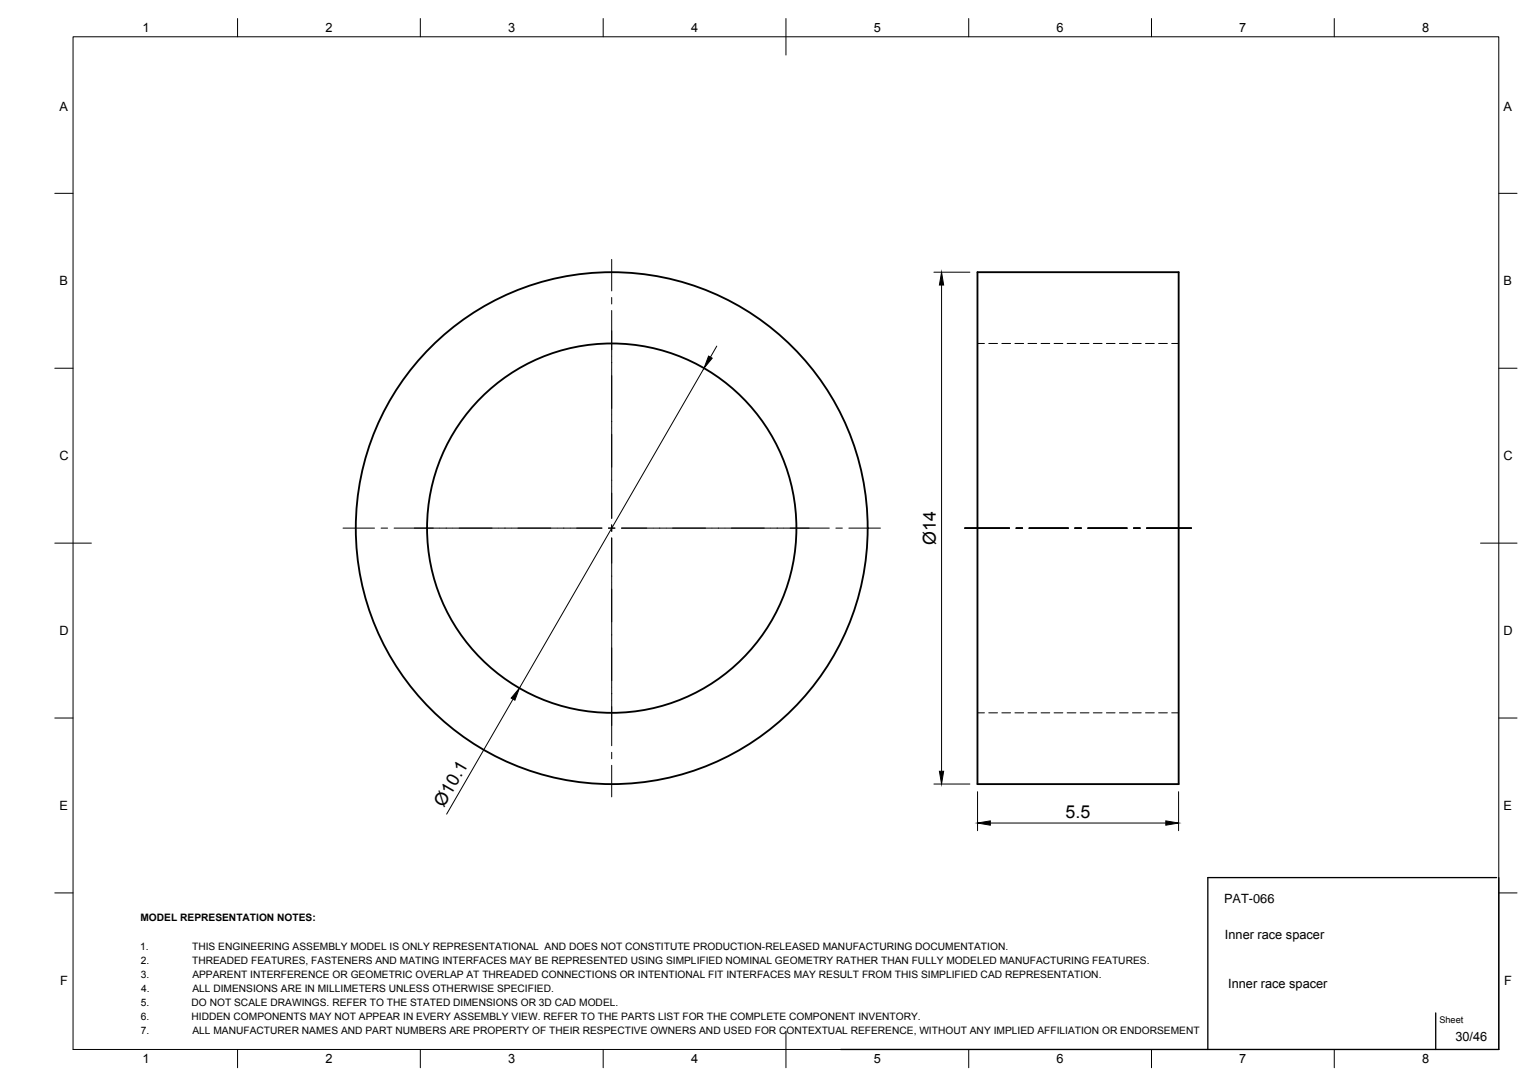
ISO-10303-21;
HEADER;
/* Generated by software containing ST-Developer
 * from STEP Tools, Inc. (www.steptools.com) 
 */

FILE_DESCRIPTION(
/* description */ ('Lever-operated bar clamp (toggle)'),
/* implementation_level */ '2;1');

FILE_NAME(
/* name */ 'Inner race spacer.step',
/* time_stamp */ '2026-10-28T03:25:02-07:00',
/* author */ (''),
/* organization */ (''),
/* preprocessor_version */ 'ST-DEVELOPER v20.2',
/* originating_system */ 'Autodesk Translation Framework v15.17.0.0',
/* authorisation */ '');

FILE_SCHEMA (('AUTOMOTIVE_DESIGN { 1 0 10303 214 3 1 1 }'));
ENDSEC;

DATA;
#10=MECHANICAL_DESIGN_GEOMETRIC_PRESENTATION_REPRESENTATION('',(#439),#12413);
#355=SHAPE_REPRESENTATION_RELATIONSHIP('SRR','None',#12597,#393);
#393=ADVANCED_BREP_SHAPE_REPRESENTATION('',(#484),#12394);
#439=STYLED_ITEM('',(#12869),#484);
#484=MANIFOLD_SOLID_BREP('Body1',#6600);
#615=FACE_BOUND('',#1676,.T.);
#616=FACE_BOUND('',#1678,.T.);
#796=PLANE('',#7588);
#797=PLANE('',#7589);
#1152=FACE_OUTER_BOUND('',#1673,.T.);
#1153=FACE_OUTER_BOUND('',#1674,.T.);
#1154=FACE_OUTER_BOUND('',#1675,.T.);
#1155=FACE_OUTER_BOUND('',#1677,.T.);
#1673=EDGE_LOOP('',(#5501,#5502,#5503,#5504));
#1674=EDGE_LOOP('',(#5505,#5506,#5507,#5508));
#1675=EDGE_LOOP('',(#5509));
#1676=EDGE_LOOP('',(#5510));
#1677=EDGE_LOOP('',(#5511));
#1678=EDGE_LOOP('',(#5512));
#2128=LINE('',#11592,#2569);
#2129=LINE('',#11598,#2570);
#2569=VECTOR('',#9261,0.505);
#2570=VECTOR('',#9268,0.7);
#2978=CIRCLE('',#7583,0.505);
#2979=CIRCLE('',#7584,0.505);
#2980=CIRCLE('',#7586,0.7);
#2981=CIRCLE('',#7587,0.7);
#3441=VERTEX_POINT('',#11589);
#3442=VERTEX_POINT('',#11591);
#3443=VERTEX_POINT('',#11595);
#3444=VERTEX_POINT('',#11597);
#4155=EDGE_CURVE('',#3441,#3441,#2978,.T.);
#4156=EDGE_CURVE('',#3441,#3442,#2128,.T.);
#4157=EDGE_CURVE('',#3442,#3442,#2979,.T.);
#4158=EDGE_CURVE('',#3443,#3443,#2980,.T.);
#4159=EDGE_CURVE('',#3443,#3444,#2129,.T.);
#4160=EDGE_CURVE('',#3444,#3444,#2981,.T.);
#5501=ORIENTED_EDGE('',*,*,#4155,.F.);
#5502=ORIENTED_EDGE('',*,*,#4156,.T.);
#5503=ORIENTED_EDGE('',*,*,#4157,.T.);
#5504=ORIENTED_EDGE('',*,*,#4156,.F.);
#5505=ORIENTED_EDGE('',*,*,#4158,.F.);
#5506=ORIENTED_EDGE('',*,*,#4159,.T.);
#5507=ORIENTED_EDGE('',*,*,#4160,.T.);
#5508=ORIENTED_EDGE('',*,*,#4159,.F.);
#5509=ORIENTED_EDGE('',*,*,#4158,.T.);
#5510=ORIENTED_EDGE('',*,*,#4155,.T.);
#5511=ORIENTED_EDGE('',*,*,#4160,.F.);
#5512=ORIENTED_EDGE('',*,*,#4157,.F.);
#6123=CYLINDRICAL_SURFACE('',#7582,0.505);
#6124=CYLINDRICAL_SURFACE('',#7585,0.7);
#6427=ADVANCED_FACE('',(#1152),#6123,.F.);
#6428=ADVANCED_FACE('',(#1153),#6124,.T.);
#6429=ADVANCED_FACE('',(#1154,#615),#796,.T.);
#6430=ADVANCED_FACE('',(#1155,#616),#797,.F.);
#6600=CLOSED_SHELL('',(#6427,#6428,#6429,#6430));
#7581=AXIS2_PLACEMENT_3D('',#11587,#9255,#9256);
#7582=AXIS2_PLACEMENT_3D('',#11588,#9257,#9258);
#7583=AXIS2_PLACEMENT_3D('',#11590,#9259,#9260);
#7584=AXIS2_PLACEMENT_3D('',#11593,#9262,#9263);
#7585=AXIS2_PLACEMENT_3D('',#11594,#9264,#9265);
#7586=AXIS2_PLACEMENT_3D('',#11596,#9266,#9267);
#7587=AXIS2_PLACEMENT_3D('',#11599,#9269,#9270);
#7588=AXIS2_PLACEMENT_3D('',#11600,#9271,#9272);
#7589=AXIS2_PLACEMENT_3D('',#11601,#9273,#9274);
#9255=DIRECTION('axis',(0.,0.,1.));
#9256=DIRECTION('refdir',(1.,0.,0.));
#9257=DIRECTION('center_axis',(0.,1.,0.));
#9258=DIRECTION('ref_axis',(1.,0.,0.));
#9259=DIRECTION('center_axis',(0.,-1.,0.));
#9260=DIRECTION('ref_axis',(1.,0.,0.));
#9261=DIRECTION('',(0.,-1.,0.));
#9262=DIRECTION('center_axis',(0.,-1.,0.));
#9263=DIRECTION('ref_axis',(1.,0.,0.));
#9264=DIRECTION('center_axis',(0.,1.,0.));
#9265=DIRECTION('ref_axis',(1.,0.,0.));
#9266=DIRECTION('center_axis',(0.,1.,0.));
#9267=DIRECTION('ref_axis',(1.,0.,0.));
#9268=DIRECTION('',(0.,-1.,0.));
#9269=DIRECTION('center_axis',(0.,1.,0.));
#9270=DIRECTION('ref_axis',(1.,0.,0.));
#9271=DIRECTION('center_axis',(0.,1.,0.));
#9272=DIRECTION('ref_axis',(1.,0.,0.));
#9273=DIRECTION('center_axis',(0.,1.,0.));
#9274=DIRECTION('ref_axis',(1.,0.,0.));
#11587=CARTESIAN_POINT('',(0.,0.,0.));
#11588=CARTESIAN_POINT('Origin',(-4.,0.45,11.));
#11589=CARTESIAN_POINT('',(-4.505,1.,11.));
#11590=CARTESIAN_POINT('Origin',(-4.,1.,11.));
#11591=CARTESIAN_POINT('',(-4.505,0.45,11.));
#11592=CARTESIAN_POINT('',(-4.505,0.45,11.));
#11593=CARTESIAN_POINT('Origin',(-4.,0.45,11.));
#11594=CARTESIAN_POINT('Origin',(-4.,0.45,11.));
#11595=CARTESIAN_POINT('',(-4.7,1.,11.));
#11596=CARTESIAN_POINT('Origin',(-4.,1.,11.));
#11597=CARTESIAN_POINT('',(-4.7,0.45,11.));
#11598=CARTESIAN_POINT('',(-4.7,0.45,11.));
#11599=CARTESIAN_POINT('Origin',(-4.,0.45,11.));
#11600=CARTESIAN_POINT('Origin',(-4.,1.,11.));
#11601=CARTESIAN_POINT('Origin',(-4.,0.45,11.));
#12348=UNCERTAINTY_MEASURE_WITH_UNIT(LENGTH_MEASURE(0.001),#12414,
'DISTANCE_ACCURACY_VALUE',
'Maximum model space distance between geometric entities at asserted c
onnectivities');
#12367=UNCERTAINTY_MEASURE_WITH_UNIT(LENGTH_MEASURE(0.001),#12414,
'DISTANCE_ACCURACY_VALUE',
'Maximum model space distance between geometric entities at asserted c
onnectivities');
#12394=(
GEOMETRIC_REPRESENTATION_CONTEXT(3)
GLOBAL_UNCERTAINTY_ASSIGNED_CONTEXT((#12348))
GLOBAL_UNIT_ASSIGNED_CONTEXT((#12414,#12416,#12417))
REPRESENTATION_CONTEXT('','3D')
);
#12413=(
GEOMETRIC_REPRESENTATION_CONTEXT(3)
GLOBAL_UNCERTAINTY_ASSIGNED_CONTEXT((#12367))
GLOBAL_UNIT_ASSIGNED_CONTEXT((#12414,#12416,#12417))
REPRESENTATION_CONTEXT('','3D')
);
#12414=(
LENGTH_UNIT()
NAMED_UNIT(*)
SI_UNIT(.CENTI.,.METRE.)
);
#12416=(
NAMED_UNIT(*)
PLANE_ANGLE_UNIT()
SI_UNIT($,.RADIAN.)
);
#12417=(
NAMED_UNIT(*)
SI_UNIT($,.STERADIAN.)
SOLID_ANGLE_UNIT()
);
#12444=SHAPE_DEFINITION_REPRESENTATION(#12496,#12597);
#12496=PRODUCT_DEFINITION_SHAPE('',$,#12643);
#12597=SHAPE_REPRESENTATION('',(#7581),#12394);
#12616=PRODUCT_DEFINITION_CONTEXT('part definition',#12753,'design');
#12643=PRODUCT_DEFINITION('Inner race spacer','Inner race spacer',#12688,
#12616);
#12688=PRODUCT_DEFINITION_FORMATION('',$,#12781);
#12753=APPLICATION_CONTEXT(
'Core Data for Automotive Mechanical Design Process');
#12754=PRODUCT_CONTEXT('part definition',#12753,'mechanical');
#12781=PRODUCT('Inner race spacer','Inner race spacer',
'Inner race spacer',(#12754));
#12863=COLOUR_RGB('Grey',0.48,0.52,0.57);
#12864=FILL_AREA_STYLE_COLOUR('',#12863);
#12865=FILL_AREA_STYLE('',(#12864));
#12866=SURFACE_STYLE_FILL_AREA(#12865);
#12867=SURFACE_SIDE_STYLE('',(#12866));
#12868=SURFACE_STYLE_USAGE(.BOTH.,#12867);
#12869=PRESENTATION_STYLE_ASSIGNMENT((#12868));
ENDSEC;
END-ISO-10303-21;
